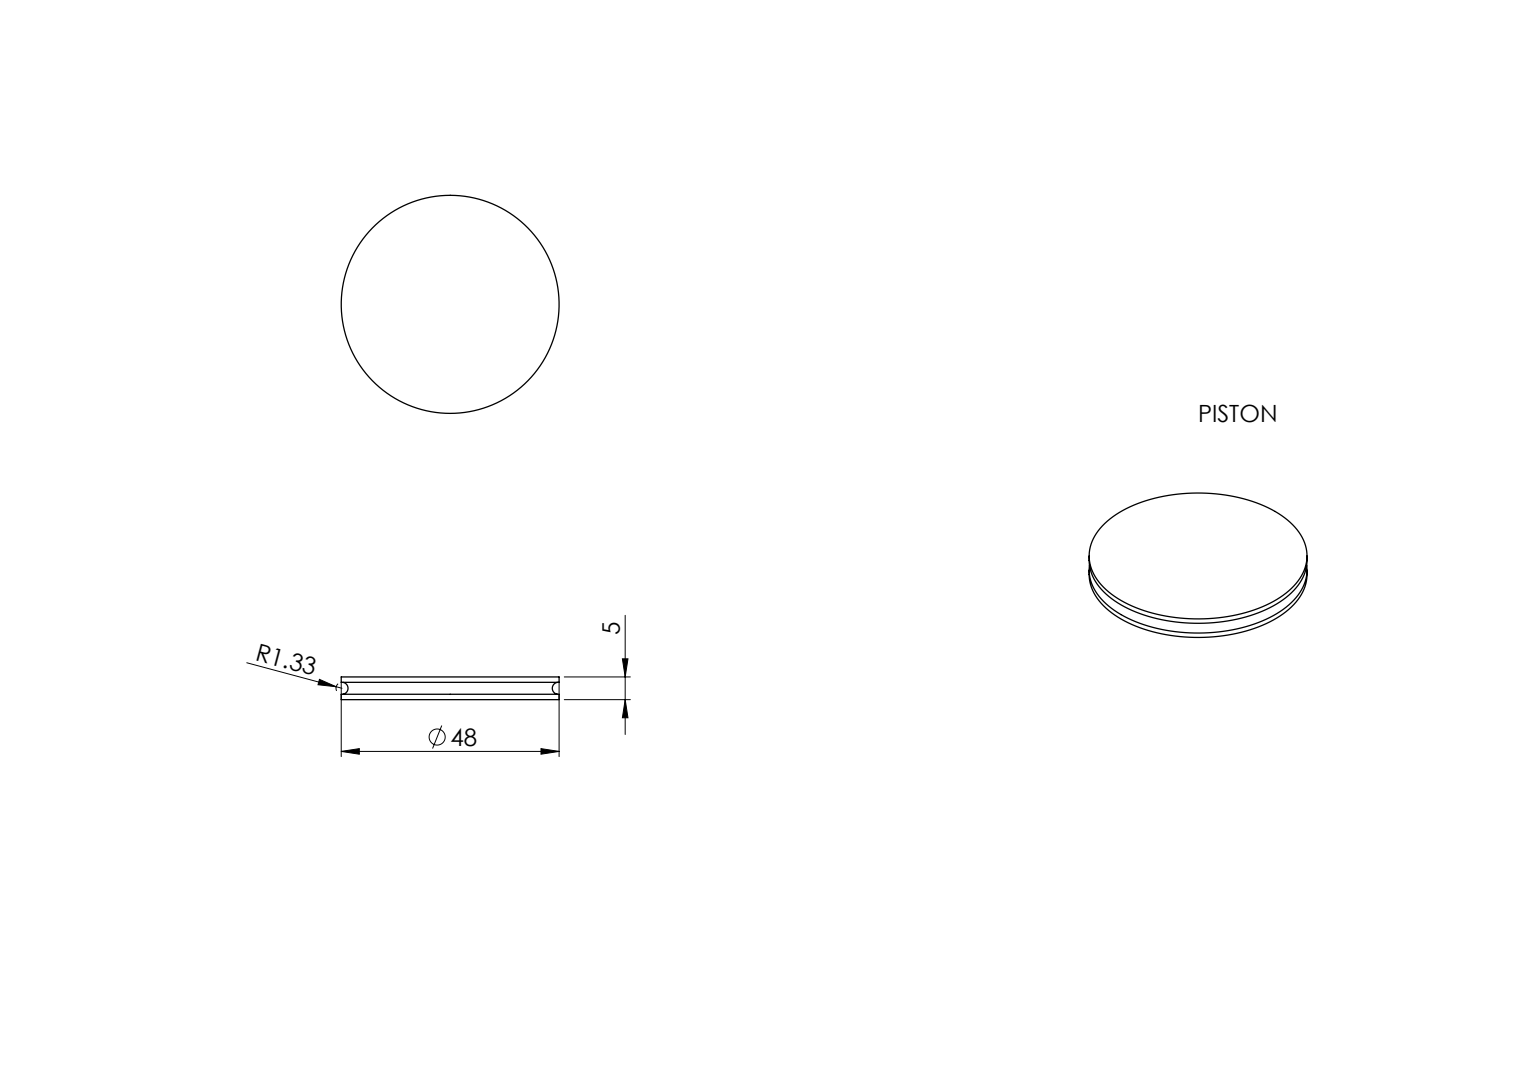
ISO-10303-21;
HEADER;
FILE_DESCRIPTION (('STEP AP214'),
    '1' );
FILE_NAME ('piston.step',
    '2026-10-24T15:06:47',
    ( '' ),
    ( '' ),
    'SwSTEP 2.0',
    'SolidWorks 2026',
    '' );
FILE_SCHEMA (( 'AUTOMOTIVE_DESIGN' ));
ENDSEC;

DATA;
#2=CARTESIAN_POINT ( 'NONE',  ( 0.000000000000000000, 72.50000000000001421, 0.000000000000000000 ) ) ;
#10=FILL_AREA_STYLE_COLOUR ( '', #10270 ) ;
#26=VERTEX_POINT ( 'NONE', #3950 ) ;
#50=AXIS2_PLACEMENT_3D ( 'NONE', #9695, #1591, #1737 ) ;
#62=FILL_AREA_STYLE ('',( #10 ) ) ;
#177=SHAPE_REPRESENTATION ( 'piston', ( #5055 ), #738 ) ;
#247=CARTESIAN_POINT ( 'NONE',  ( 0.000000000000000000, 73.81339255365637086, 0.000000000000000000 ) ) ;
#277=ORIENTED_EDGE ( 'NONE', *, *, #5688, .F. ) ;
#283=DIRECTION ( 'NONE',  ( 8.881784197001252323E-16, 0.000000000000000000, 1.000000000000000000 ) ) ;
#310=EDGE_CURVE ( 'NONE', #1877, #7747, #8787, .T. ) ;
#387=CARTESIAN_POINT ( 'NONE',  ( 2.939152317953647500E-15, 73.81339255365637086, -23.99999999999999645 ) ) ;
#440=AXIS2_PLACEMENT_3D ( 'NONE', #5333, #6948, #1461 ) ;
#452=CARTESIAN_POINT ( 'NONE',  ( 22.50000000000000355, 72.50000000000001421, -2.755455298081545172E-15 ) ) ;
#482=ORIENTED_EDGE ( 'NONE', *, *, #7517, .T. ) ;
#553=ADVANCED_FACE ( 'NONE', ( #6389 ), #3451, .F. ) ;
#580=CIRCLE ( 'NONE', #7259, 23.99999999999999645 ) ;
#600=VERTEX_POINT ( 'NONE', #6490 ) ;
#615=AXIS2_PLACEMENT_3D ( 'NONE', #4071, #9758, #8930 ) ;
#664=DIRECTION ( 'NONE',  ( -0.000000000000000000, 1.000000000000000000, -0.000000000000000000 ) ) ;
#710=FACE_OUTER_BOUND ( 'NONE', #8929, .T. ) ;
#738=( GEOMETRIC_REPRESENTATION_CONTEXT ( 3 ) GLOBAL_UNCERTAINTY_ASSIGNED_CONTEXT ( ( #10215 ) ) GLOBAL_UNIT_ASSIGNED_CONTEXT ( ( #2949, #3785, #10172 ) ) REPRESENTATION_CONTEXT ( 'NONE', 'WORKASPACE' ) );
#753=CIRCLE ( 'NONE', #7274, 23.99999999999999645 ) ;
#782=DIRECTION ( 'NONE',  ( -0.000000000000000000, 1.000000000000000000, -0.000000000000000000 ) ) ;
#784=ADVANCED_FACE ( 'NONE', ( #710 ), #3851, .T. ) ;
#858=EDGE_CURVE ( 'NONE', #7847, #7747, #5465, .T. ) ;
#887=EDGE_CURVE ( 'NONE', #1976, #26, #7608, .T. ) ;
#901=SHAPE_REPRESENTATION_RELATIONSHIP ( 'NONE' , 'NONE' ,  #177, #3150 ) ;
#953=DIRECTION ( 'NONE',  ( 1.000000000000000000, 0.000000000000000000, 0.000000000000000000 ) ) ;
#1070=CARTESIAN_POINT ( 'NONE',  ( 0.000000000000000000, 73.81339255365637086, 0.000000000000000000 ) ) ;
#1076=CARTESIAN_POINT ( 'NONE',  ( -22.50000000000000355, 72.50000000000001421, 0.000000000000000000 ) ) ;
#1138=CIRCLE ( 'NONE', #6996, 23.99999999999999645 ) ;
#1416=UNCERTAINTY_MEASURE_WITH_UNIT (LENGTH_MEASURE( 1.000000000000000082E-05 ), #8634, 'distance_accuracy_value', 'NONE');
#1421=PRODUCT_DEFINITION_SHAPE ( 'NONE', 'NONE',  #3149 ) ;
#1458=( NAMED_UNIT ( * ) PLANE_ANGLE_UNIT ( ) SI_UNIT ( $, .RADIAN. ) );
#1461=DIRECTION ( 'NONE',  ( -1.000000000000000000, 0.000000000000000000, 1.224646799147352961E-16 ) ) ;
#1480=SURFACE_STYLE_FILL_AREA ( #62 ) ;
#1509=ORIENTED_EDGE ( 'NONE', *, *, #310, .F. ) ;
#1546=CARTESIAN_POINT ( 'NONE',  ( 0.000000000000000000, 75.00000000000001421, 0.000000000000000000 ) ) ;
#1550=ORIENTED_EDGE ( 'NONE', *, *, #4131, .T. ) ;
#1570=( GEOMETRIC_REPRESENTATION_CONTEXT ( 3 ) GLOBAL_UNCERTAINTY_ASSIGNED_CONTEXT ( ( #2145 ) ) GLOBAL_UNIT_ASSIGNED_CONTEXT ( ( #2268, #3164, #9494 ) ) REPRESENTATION_CONTEXT ( 'NONE', 'WORKASPACE' ) );
#1591=DIRECTION ( 'NONE',  ( 0.000000000000000000, -1.000000000000000000, 0.000000000000000000 ) ) ;
#1601=LINE ( 'NONE', #7991, #10153 ) ;
#1631=ORIENTED_EDGE ( 'NONE', *, *, #5530, .F. ) ;
#1685=DIRECTION ( 'NONE',  ( 0.000000000000000000, -1.000000000000000000, 0.000000000000000000 ) ) ;
#1737=DIRECTION ( 'NONE',  ( 0.000000000000000000, 0.000000000000000000, -1.000000000000000000 ) ) ;
#1749=ORIENTED_EDGE ( 'NONE', *, *, #5688, .T. ) ;
#1765=EDGE_CURVE ( 'NONE', #8002, #10148, #10057, .T. ) ;
#1877=VERTEX_POINT ( 'NONE', #387 ) ;
#1880=EDGE_CURVE ( 'NONE', #2411, #4835, #5392, .T. ) ;
#1885=ORIENTED_EDGE ( 'NONE', *, *, #7543, .T. ) ;
#1897=EDGE_CURVE ( 'NONE', #4746, #8517, #7219, .T. ) ;
#1957=DIRECTION ( 'NONE',  ( -0.000000000000000000, -1.000000000000000000, 0.000000000000000000 ) ) ;
#1976=VERTEX_POINT ( 'NONE', #2173 ) ;
#2004=DIRECTION ( 'NONE',  ( -1.000000000000000000, 0.000000000000000000, 0.000000000000000000 ) ) ;
#2016=CIRCLE ( 'NONE', #6212, 22.50000000000000355 ) ;
#2040=AXIS2_PLACEMENT_3D ( 'NONE', #2702, #1957, #2004 ) ;
#2057=MECHANICAL_DESIGN_GEOMETRIC_PRESENTATION_REPRESENTATION('',(#9429),#1570);
#2145=UNCERTAINTY_MEASURE_WITH_UNIT (LENGTH_MEASURE( 1.000000000000000082E-05 ), #2268, 'distance_accuracy_value', 'NONE');
#2161=EDGE_LOOP ( 'NONE', ( #1509, #3667, #482, #1885, #5735 ) ) ;
#2173=CARTESIAN_POINT ( 'NONE',  ( -24.00000000000000711, 71.18660744634364335, 0.000000000000000000 ) ) ;
#2196=PRODUCT_CONTEXT ( 'NONE', #7453, 'mechanical' ) ;
#2268=( LENGTH_UNIT ( ) NAMED_UNIT ( * ) SI_UNIT ( .MILLI., .METRE. ) );
#2320=EDGE_CURVE ( 'NONE', #2411, #600, #3373, .T. ) ;
#2345=DIRECTION ( 'NONE',  ( 0.000000000000000000, 0.000000000000000000, 1.000000000000000000 ) ) ;
#2375=ADVANCED_FACE ( 'NONE', ( #4272 ), #5566, .F. ) ;
#2411=VERTEX_POINT ( 'NONE', #1076 ) ;
#2441=AXIS2_PLACEMENT_3D ( 'NONE', #6592, #8319, #953 ) ;
#2478=CARTESIAN_POINT ( 'NONE',  ( 0.000000000000000000, 73.81339255365637086, 0.000000000000000000 ) ) ;
#2562=DIRECTION ( 'NONE',  ( -1.000000000000000000, 0.000000000000000000, 0.000000000000000000 ) ) ;
#2596=TOROIDAL_SURFACE ( 'NONE', #5935, 23.82500000000000284, 1.324999999999999956 ) ;
#2702=CARTESIAN_POINT ( 'NONE',  ( 0.000000000000000000, 72.50000000000001421, 0.000000000000000000 ) ) ;
#2722=CARTESIAN_POINT ( 'NONE',  ( 2.939152317953647500E-15, 70.00000000000000000, -23.99999999999999645 ) ) ;
#2812=DIRECTION ( 'NONE',  ( 0.000000000000000000, 1.000000000000000000, -0.000000000000000000 ) ) ;
#2913=PLANE ( 'NONE',  #8914 ) ;
#2923=EDGE_LOOP ( 'NONE', ( #7895, #6101 ) ) ;
#2949=( LENGTH_UNIT ( ) NAMED_UNIT ( * ) SI_UNIT ( .MILLI., .METRE. ) );
#2987=AXIS2_PLACEMENT_3D ( 'NONE', #2478, #9690, #8908 ) ;
#3019=ORIENTED_EDGE ( 'NONE', *, *, #1880, .F. ) ;
#3075=CARTESIAN_POINT ( 'NONE',  ( 0.000000000000000000, 71.18660744634364335, 0.000000000000000000 ) ) ;
#3129=DIRECTION ( 'NONE',  ( 0.000000000000000000, 0.000000000000000000, 1.000000000000000000 ) ) ;
#3138=DIRECTION ( 'NONE',  ( -1.000000000000000000, 0.000000000000000000, 1.224646799147352961E-16 ) ) ;
#3149=PRODUCT_DEFINITION ( 'UNKNOWN', '', #5131, #9255 ) ;
#3150=ADVANCED_BREP_SHAPE_REPRESENTATION ( '', ( #6259, #5055 ), #738 ) ;
#3164=( NAMED_UNIT ( * ) PLANE_ANGLE_UNIT ( ) SI_UNIT ( $, .RADIAN. ) );
#3235=CIRCLE ( 'NONE', #50, 23.99999999999999645 ) ;
#3253=DIRECTION ( 'NONE',  ( -1.000000000000000000, 0.000000000000000000, 0.000000000000000000 ) ) ;
#3280=CIRCLE ( 'NONE', #9774, 1.324999999999999734 ) ;
#3333=CARTESIAN_POINT ( 'NONE',  ( 0.000000000000000000, 70.00000000000000000, 23.99999999999999645 ) ) ;
#3337=EDGE_CURVE ( 'NONE', #7747, #7847, #3235, .T. ) ;
#3342=FACE_OUTER_BOUND ( 'NONE', #5022, .T. ) ;
#3373=CIRCLE ( 'NONE', #7726, 1.324999999999999734 ) ;
#3385=DIRECTION ( 'NONE',  ( -0.000000000000000000, -1.000000000000000000, 0.000000000000000000 ) ) ;
#3393=ORIENTED_EDGE ( 'NONE', *, *, #3520, .T. ) ;
#3451=TOROIDAL_SURFACE ( 'NONE', #9300, 23.82500000000000284, 1.324999999999999956 ) ;
#3520=EDGE_CURVE ( 'NONE', #4835, #2411, #2016, .T. ) ;
#3524=DIRECTION ( 'NONE',  ( -0.000000000000000000, -1.000000000000000000, 0.000000000000000000 ) ) ;
#3594=AXIS2_PLACEMENT_3D ( 'NONE', #247, #2812, #5797 ) ;
#3599=PLANE ( 'NONE',  #10350 ) ;
#3654=CARTESIAN_POINT ( 'NONE',  ( 0.000000000000000000, 75.00000000000001421, 0.000000000000000000 ) ) ;
#3667=ORIENTED_EDGE ( 'NONE', *, *, #6650, .T. ) ;
#3705=DIRECTION ( 'NONE',  ( 0.000000000000000000, -0.000000000000000000, -1.000000000000000000 ) ) ;
#3733=DIRECTION ( 'NONE',  ( 0.000000000000000000, 0.000000000000000000, 1.000000000000000000 ) ) ;
#3783=AXIS2_PLACEMENT_3D ( 'NONE', #1546, #10130, #10243 ) ;
#3785=( NAMED_UNIT ( * ) PLANE_ANGLE_UNIT ( ) SI_UNIT ( $, .RADIAN. ) );
#3787=DIRECTION ( 'NONE',  ( 0.000000000000000000, 0.000000000000000000, 1.000000000000000000 ) ) ;
#3809=ORIENTED_EDGE ( 'NONE', *, *, #4131, .F. ) ;
#3816=DIRECTION ( 'NONE',  ( -0.000000000000000000, 1.000000000000000000, -0.000000000000000000 ) ) ;
#3851=CYLINDRICAL_SURFACE ( 'NONE', #10131, 23.99999999999999645 ) ;
#3946=VECTOR ( 'NONE', #9820, 1000.000000000000000 ) ;
#3950=CARTESIAN_POINT ( 'NONE',  ( 2.939152317953647500E-15, 71.18660744634364335, -23.99999999999999645 ) ) ;
#3962=TOROIDAL_SURFACE ( 'NONE', #5960, 23.82500000000000284, 1.324999999999999956 ) ;
#3965=CARTESIAN_POINT ( 'NONE',  ( 0.000000000000000000, 72.50000000000001421, 0.000000000000000000 ) ) ;
#4071=CARTESIAN_POINT ( 'NONE',  ( 0.000000000000000000, 70.00000000000000000, 0.000000000000000000 ) ) ;
#4096=CIRCLE ( 'NONE', #8106, 23.99999999999999645 ) ;
#4115=EDGE_CURVE ( 'NONE', #8517, #1976, #580, .T. ) ;
#4131=EDGE_CURVE ( 'NONE', #26, #4746, #4096, .T. ) ;
#4154=DIRECTION ( 'NONE',  ( 0.000000000000000000, 0.000000000000000000, 1.000000000000000000 ) ) ;
#4262=CIRCLE ( 'NONE', #2441, 1.324999999999999734 ) ;
#4264=CYLINDRICAL_SURFACE ( 'NONE', #615, 23.99999999999999645 ) ;
#4272=FACE_OUTER_BOUND ( 'NONE', #6236, .T. ) ;
#4278=CARTESIAN_POINT ( 'NONE',  ( 0.000000000000000000, 72.50000000000001421, 0.000000000000000000 ) ) ;
#4286=CARTESIAN_POINT ( 'NONE',  ( 0.000000000000000000, 73.81339255365637086, 0.000000000000000000 ) ) ;
#4314=DIRECTION ( 'NONE',  ( 0.000000000000000000, 1.000000000000000000, -0.000000000000000000 ) ) ;
#4352=STYLED_ITEM('',(#10394),#6259);
#4369=DIRECTION ( 'NONE',  ( 0.000000000000000000, -0.000000000000000000, -1.000000000000000000 ) ) ;
#4405=EDGE_CURVE ( 'NONE', #6757, #6493, #753, .T. ) ;
#4412=EDGE_LOOP ( 'NONE', ( #6624, #4996, #1550, #5367, #6893 ) ) ;
#4416=DIRECTION ( 'NONE',  ( -0.000000000000000000, -1.000000000000000000, 0.000000000000000000 ) ) ;
#4506=EDGE_LOOP ( 'NONE', ( #9987, #1631, #4846, #6958, #5378 ) ) ;
#4524=FACE_OUTER_BOUND ( 'NONE', #4412, .T. ) ;
#4583=DIRECTION ( 'NONE',  ( 0.000000000000000000, 0.000000000000000000, 1.000000000000000000 ) ) ;
#4622=CARTESIAN_POINT ( 'NONE',  ( 0.000000000000000000, 71.18660744634364335, 0.000000000000000000 ) ) ;
#4650=CYLINDRICAL_SURFACE ( 'NONE', #9705, 23.99999999999999645 ) ;
#4746=VERTEX_POINT ( 'NONE', #9036 ) ;
#4749=DIRECTION ( 'NONE',  ( -1.224646799147353207E-16, 0.000000000000000000, -1.000000000000000000 ) ) ;
#4835=VERTEX_POINT ( 'NONE', #452 ) ;
#4846=ORIENTED_EDGE ( 'NONE', *, *, #5943, .T. ) ;
#4951=AXIS2_PLACEMENT_3D ( 'NONE', #7719, #5987, #4583 ) ;
#4996=ORIENTED_EDGE ( 'NONE', *, *, #8566, .T. ) ;
#5022=EDGE_LOOP ( 'NONE', ( #1749, #6205, #6376, #3809, #9862 ) ) ;
#5055=AXIS2_PLACEMENT_3D ( 'NONE', #9842, #4154, #9744 ) ;
#5079=ORIENTED_EDGE ( 'NONE', *, *, #7948, .F. ) ;
#5131=PRODUCT_DEFINITION_FORMATION_WITH_SPECIFIED_SOURCE ( 'ANY', '', #5693, .NOT_KNOWN. ) ;
#5203=AXIS2_PLACEMENT_3D ( 'NONE', #4286, #6741, #7470 ) ;
#5251=EDGE_LOOP ( 'NONE', ( #3019, #9847, #8245, #8860, #5079 ) ) ;
#5252=CARTESIAN_POINT ( 'NONE',  ( 2.939152317953647500E-15, 75.00000000000001421, -23.99999999999999645 ) ) ;
#5311=EDGE_CURVE ( 'NONE', #10148, #1877, #7113, .T. ) ;
#5333=CARTESIAN_POINT ( 'NONE',  ( 23.82500000000000284, 72.50000000000001421, -2.917720998968569322E-15 ) ) ;
#5367=ORIENTED_EDGE ( 'NONE', *, *, #1897, .T. ) ;
#5378=ORIENTED_EDGE ( 'NONE', *, *, #887, .T. ) ;
#5392=CIRCLE ( 'NONE', #6553, 22.50000000000000355 ) ;
#5401=ORIENTED_EDGE ( 'NONE', *, *, #2320, .F. ) ;
#5465=CIRCLE ( 'NONE', #3783, 23.99999999999999645 ) ;
#5467=PRESENTATION_STYLE_ASSIGNMENT (( #9638 ) ) ;
#5468=DIRECTION ( 'NONE',  ( -0.000000000000000000, -1.000000000000000000, 0.000000000000000000 ) ) ;
#5491=EDGE_CURVE ( 'NONE', #4746, #4835, #3280, .T. ) ;
#5519=CARTESIAN_POINT ( 'NONE',  ( 0.000000000000000000, 70.00000000000000000, 0.000000000000000000 ) ) ;
#5530=EDGE_CURVE ( 'NONE', #6493, #6757, #10126, .T. ) ;
#5564=SURFACE_SIDE_STYLE ('',( #1480 ) ) ;
#5566=TOROIDAL_SURFACE ( 'NONE', #2040, 23.82500000000000284, 1.324999999999999956 ) ;
#5642=VECTOR ( 'NONE', #782, 1000.000000000000000 ) ;
#5644=DIRECTION ( 'NONE',  ( 0.000000000000000000, -1.000000000000000000, 0.000000000000000000 ) ) ;
#5688=EDGE_CURVE ( 'NONE', #1976, #2411, #4262, .T. ) ;
#5693=PRODUCT ( 'piston', 'piston', '', ( #2196 ) ) ;
#5694=ORIENTED_EDGE ( 'NONE', *, *, #4115, .F. ) ;
#5735=ORIENTED_EDGE ( 'NONE', *, *, #858, .T. ) ;
#5797=DIRECTION ( 'NONE',  ( -8.881784197001252323E-16, 0.000000000000000000, -1.000000000000000000 ) ) ;
#5852=MECHANICAL_DESIGN_GEOMETRIC_PRESENTATION_REPRESENTATION('',(#4352),#7037);
#5933=ADVANCED_FACE ( 'NONE', ( #3342 ), #2596, .F. ) ;
#5935=AXIS2_PLACEMENT_3D ( 'NONE', #4278, #3385, #2562 ) ;
#5943=EDGE_CURVE ( 'NONE', #6493, #8517, #9040, .T. ) ;
#5960=AXIS2_PLACEMENT_3D ( 'NONE', #6197, #8444, #10185 ) ;
#5987=DIRECTION ( 'NONE',  ( -0.000000000000000000, 1.000000000000000000, -0.000000000000000000 ) ) ;
#6023=ORIENTED_EDGE ( 'NONE', *, *, #5530, .T. ) ;
#6094=CYLINDRICAL_SURFACE ( 'NONE', #4951, 23.99999999999999645 ) ;
#6096=DIRECTION ( 'NONE',  ( 0.000000000000000000, -1.000000000000000000, 0.000000000000000000 ) ) ;
#6101=ORIENTED_EDGE ( 'NONE', *, *, #3337, .F. ) ;
#6157=VECTOR ( 'NONE', #9808, 1000.000000000000000 ) ;
#6191=CARTESIAN_POINT ( 'NONE',  ( 0.000000000000000000, 70.00000000000000000, 23.99999999999999645 ) ) ;
#6197=CARTESIAN_POINT ( 'NONE',  ( 0.000000000000000000, 72.50000000000001421, 0.000000000000000000 ) ) ;
#6205=ORIENTED_EDGE ( 'NONE', *, *, #1880, .T. ) ;
#6212=AXIS2_PLACEMENT_3D ( 'NONE', #3965, #7151, #9564 ) ;
#6236=EDGE_LOOP ( 'NONE', ( #6658, #9594, #10061, #8627, #5401 ) ) ;
#6259=MANIFOLD_SOLID_BREP ( 'Cavity1', #10150 ) ;
#6269=ADVANCED_FACE ( 'NONE', ( #6426 ), #4650, .T. ) ;
#6376=ORIENTED_EDGE ( 'NONE', *, *, #5491, .F. ) ;
#6389=FACE_OUTER_BOUND ( 'NONE', #5251, .T. ) ;
#6413=ADVANCED_FACE ( 'NONE', ( #9080 ), #4264, .T. ) ;
#6426=FACE_OUTER_BOUND ( 'NONE', #2161, .T. ) ;
#6490=CARTESIAN_POINT ( 'NONE',  ( -24.00000000000000711, 73.81339255365637086, 0.000000000000000000 ) ) ;
#6493=VERTEX_POINT ( 'NONE', #6191 ) ;
#6540=ORIENTED_EDGE ( 'NONE', *, *, #1765, .T. ) ;
#6553=AXIS2_PLACEMENT_3D ( 'NONE', #7601, #3524, #7441 ) ;
#6592=CARTESIAN_POINT ( 'NONE',  ( -23.82500000000000284, 72.50000000000001421, 0.000000000000000000 ) ) ;
#6624=ORIENTED_EDGE ( 'NONE', *, *, #4405, .F. ) ;
#6650=EDGE_CURVE ( 'NONE', #1877, #600, #7475, .T. ) ;
#6658=ORIENTED_EDGE ( 'NONE', *, *, #3520, .F. ) ;
#6741=DIRECTION ( 'NONE',  ( 0.000000000000000000, 1.000000000000000000, -0.000000000000000000 ) ) ;
#6757=VERTEX_POINT ( 'NONE', #2722 ) ;
#6770=ORIENTED_EDGE ( 'NONE', *, *, #310, .T. ) ;
#6826=DIRECTION ( 'NONE',  ( 1.000000000000000000, 0.000000000000000000, 0.000000000000000000 ) ) ;
#6834=DIRECTION ( 'NONE',  ( 0.000000000000000000, -1.000000000000000000, 0.000000000000000000 ) ) ;
#6893=ORIENTED_EDGE ( 'NONE', *, *, #5943, .F. ) ;
#6895=SHAPE_DEFINITION_REPRESENTATION ( #1421, #177 ) ;
#6911=EDGE_LOOP ( 'NONE', ( #6023, #9540 ) ) ;
#6948=DIRECTION ( 'NONE',  ( -1.224646799147353207E-16, 0.000000000000000000, -1.000000000000000000 ) ) ;
#6958=ORIENTED_EDGE ( 'NONE', *, *, #4115, .T. ) ;
#6996=AXIS2_PLACEMENT_3D ( 'NONE', #1070, #4314, #8981 ) ;
#7037=( GEOMETRIC_REPRESENTATION_CONTEXT ( 3 ) GLOBAL_UNCERTAINTY_ASSIGNED_CONTEXT ( ( #1416 ) ) GLOBAL_UNIT_ASSIGNED_CONTEXT ( ( #8634, #1458, #7842 ) ) REPRESENTATION_CONTEXT ( 'NONE', 'WORKASPACE' ) );
#7113=CIRCLE ( 'NONE', #3594, 23.99999999999999645 ) ;
#7121=DIRECTION ( 'NONE',  ( -0.000000000000000000, -1.000000000000000000, 0.000000000000000000 ) ) ;
#7151=DIRECTION ( 'NONE',  ( -0.000000000000000000, -1.000000000000000000, 0.000000000000000000 ) ) ;
#7155=DIRECTION ( 'NONE',  ( 0.000000000000000000, 0.000000000000000000, -1.000000000000000000 ) ) ;
#7219=CIRCLE ( 'NONE', #8898, 23.99999999999999645 ) ;
#7257=ORIENTED_EDGE ( 'NONE', *, *, #5311, .T. ) ;
#7259=AXIS2_PLACEMENT_3D ( 'NONE', #4622, #8658, #3787 ) ;
#7274=AXIS2_PLACEMENT_3D ( 'NONE', #5519, #1685, #8072 ) ;
#7286=AXIS2_PLACEMENT_3D ( 'NONE', #3075, #9401, #8621 ) ;
#7339=ADVANCED_FACE ( 'NONE', ( #7732 ), #3599, .F. ) ;
#7441=DIRECTION ( 'NONE',  ( 0.000000000000000000, 0.000000000000000000, -1.000000000000000000 ) ) ;
#7453=APPLICATION_CONTEXT ( 'automotive_design' ) ;
#7470=DIRECTION ( 'NONE',  ( 0.000000000000000000, 0.000000000000000000, -1.000000000000000000 ) ) ;
#7475=CIRCLE ( 'NONE', #2987, 23.99999999999999645 ) ;
#7517=EDGE_CURVE ( 'NONE', #600, #8002, #1138, .T. ) ;
#7543=EDGE_CURVE ( 'NONE', #8002, #7847, #9759, .T. ) ;
#7601=CARTESIAN_POINT ( 'NONE',  ( 0.000000000000000000, 72.50000000000001421, 0.000000000000000000 ) ) ;
#7608=CIRCLE ( 'NONE', #7286, 23.99999999999999645 ) ;
#7719=CARTESIAN_POINT ( 'NONE',  ( 0.000000000000000000, 70.00000000000000000, 0.000000000000000000 ) ) ;
#7726=AXIS2_PLACEMENT_3D ( 'NONE', #8298, #9920, #6826 ) ;
#7732=FACE_OUTER_BOUND ( 'NONE', #2923, .T. ) ;
#7747=VERTEX_POINT ( 'NONE', #5252 ) ;
#7842=( NAMED_UNIT ( * ) SI_UNIT ( $, .STERADIAN. ) SOLID_ANGLE_UNIT ( ) );
#7847=VERTEX_POINT ( 'NONE', #8307 ) ;
#7895=ORIENTED_EDGE ( 'NONE', *, *, #858, .F. ) ;
#7948=EDGE_CURVE ( 'NONE', #4835, #10148, #9302, .T. ) ;
#7951=CARTESIAN_POINT ( 'NONE',  ( 2.939152317953647500E-15, 70.00000000000000000, -23.99999999999999645 ) ) ;
#7976=ORIENTED_EDGE ( 'NONE', *, *, #1897, .F. ) ;
#7991=CARTESIAN_POINT ( 'NONE',  ( 2.939152317953647500E-15, 70.00000000000000000, -23.99999999999999645 ) ) ;
#8002=VERTEX_POINT ( 'NONE', #10032 ) ;
#8046=CARTESIAN_POINT ( 'NONE',  ( 0.000000000000000000, 70.00000000000000000, 0.000000000000000000 ) ) ;
#8072=DIRECTION ( 'NONE',  ( 0.000000000000000000, 0.000000000000000000, -1.000000000000000000 ) ) ;
#8106=AXIS2_PLACEMENT_3D ( 'NONE', #10055, #5468, #3733 ) ;
#8245=ORIENTED_EDGE ( 'NONE', *, *, #6650, .F. ) ;
#8278=AXIS2_PLACEMENT_3D ( 'NONE', #8046, #5644, #7155 ) ;
#8298=CARTESIAN_POINT ( 'NONE',  ( -23.82500000000000284, 72.50000000000001421, 0.000000000000000000 ) ) ;
#8307=CARTESIAN_POINT ( 'NONE',  ( 0.000000000000000000, 75.00000000000001421, 23.99999999999999645 ) ) ;
#8319=DIRECTION ( 'NONE',  ( 0.000000000000000000, 0.000000000000000000, 1.000000000000000000 ) ) ;
#8378=ADVANCED_FACE ( 'NONE', ( #4524 ), #6094, .T. ) ;
#8444=DIRECTION ( 'NONE',  ( -0.000000000000000000, -1.000000000000000000, 0.000000000000000000 ) ) ;
#8517=VERTEX_POINT ( 'NONE', #10352 ) ;
#8548=APPLICATION_CONTEXT ( 'automotive_design' ) ;
#8566=EDGE_CURVE ( 'NONE', #6757, #26, #1601, .T. ) ;
#8621=DIRECTION ( 'NONE',  ( 0.000000000000000000, 0.000000000000000000, 1.000000000000000000 ) ) ;
#8627=ORIENTED_EDGE ( 'NONE', *, *, #7517, .F. ) ;
#8634=( LENGTH_UNIT ( ) NAMED_UNIT ( * ) SI_UNIT ( .MILLI., .METRE. ) );
#8658=DIRECTION ( 'NONE',  ( -0.000000000000000000, -1.000000000000000000, 0.000000000000000000 ) ) ;
#8681=ORIENTED_EDGE ( 'NONE', *, *, #5491, .T. ) ;
#8787=LINE ( 'NONE', #7951, #5642 ) ;
#8860=ORIENTED_EDGE ( 'NONE', *, *, #5311, .F. ) ;
#8898=AXIS2_PLACEMENT_3D ( 'NONE', #9963, #4416, #283 ) ;
#8908=DIRECTION ( 'NONE',  ( 0.000000000000000000, 0.000000000000000000, -1.000000000000000000 ) ) ;
#8914=AXIS2_PLACEMENT_3D ( 'NONE', #10021, #6096, #4369 ) ;
#8926=FACE_OUTER_BOUND ( 'NONE', #9903, .T. ) ;
#8929=EDGE_LOOP ( 'NONE', ( #7257, #6770, #8948, #9224, #6540 ) ) ;
#8930=DIRECTION ( 'NONE',  ( 0.000000000000000000, 0.000000000000000000, 1.000000000000000000 ) ) ;
#8948=ORIENTED_EDGE ( 'NONE', *, *, #3337, .T. ) ;
#8981=DIRECTION ( 'NONE',  ( 0.000000000000000000, 0.000000000000000000, -1.000000000000000000 ) ) ;
#9036=CARTESIAN_POINT ( 'NONE',  ( 24.00000000000000711, 71.18660744634364335, -2.939152317953649078E-15 ) ) ;
#9040=LINE ( 'NONE', #9871, #3946 ) ;
#9080=FACE_OUTER_BOUND ( 'NONE', #4506, .T. ) ;
#9224=ORIENTED_EDGE ( 'NONE', *, *, #7543, .F. ) ;
#9255=PRODUCT_DEFINITION_CONTEXT ( 'detailed design', #8548, 'design' ) ;
#9289=CARTESIAN_POINT ( 'NONE',  ( 24.00000000000000711, 73.81339255365637086, -2.939152317953649078E-15 ) ) ;
#9300=AXIS2_PLACEMENT_3D ( 'NONE', #2, #7121, #3253 ) ;
#9302=CIRCLE ( 'NONE', #440, 1.324999999999999734 ) ;
#9401=DIRECTION ( 'NONE',  ( -0.000000000000000000, -1.000000000000000000, 0.000000000000000000 ) ) ;
#9413=CARTESIAN_POINT ( 'NONE',  ( 0.000000000000000000, 70.00000000000000000, 0.000000000000000000 ) ) ;
#9429=STYLED_ITEM ( 'NONE', ( #5467 ), #3150 ) ;
#9494=( NAMED_UNIT ( * ) SI_UNIT ( $, .STERADIAN. ) SOLID_ANGLE_UNIT ( ) );
#9540=ORIENTED_EDGE ( 'NONE', *, *, #4405, .T. ) ;
#9554=ADVANCED_FACE ( 'NONE', ( #8926 ), #3962, .F. ) ;
#9559=CARTESIAN_POINT ( 'NONE',  ( 0.000000000000000000, 70.00000000000000000, 0.000000000000000000 ) ) ;
#9564=DIRECTION ( 'NONE',  ( 0.000000000000000000, 0.000000000000000000, -1.000000000000000000 ) ) ;
#9594=ORIENTED_EDGE ( 'NONE', *, *, #7948, .T. ) ;
#9638=SURFACE_STYLE_USAGE ( .BOTH. , #5564 ) ;
#9690=DIRECTION ( 'NONE',  ( 0.000000000000000000, 1.000000000000000000, -0.000000000000000000 ) ) ;
#9695=CARTESIAN_POINT ( 'NONE',  ( 0.000000000000000000, 75.00000000000001421, 0.000000000000000000 ) ) ;
#9705=AXIS2_PLACEMENT_3D ( 'NONE', #9413, #3816, #2345 ) ;
#9744=DIRECTION ( 'NONE',  ( 1.000000000000000000, 0.000000000000000000, 0.000000000000000000 ) ) ;
#9758=DIRECTION ( 'NONE',  ( -0.000000000000000000, 1.000000000000000000, -0.000000000000000000 ) ) ;
#9759=LINE ( 'NONE', #3333, #6157 ) ;
#9774=AXIS2_PLACEMENT_3D ( 'NONE', #10305, #4749, #3138 ) ;
#9808=DIRECTION ( 'NONE',  ( -0.000000000000000000, 1.000000000000000000, -0.000000000000000000 ) ) ;
#9820=DIRECTION ( 'NONE',  ( -0.000000000000000000, 1.000000000000000000, -0.000000000000000000 ) ) ;
#9842=CARTESIAN_POINT ( 'NONE',  ( 0.000000000000000000, 0.000000000000000000, 0.000000000000000000 ) ) ;
#9847=ORIENTED_EDGE ( 'NONE', *, *, #2320, .T. ) ;
#9862=ORIENTED_EDGE ( 'NONE', *, *, #887, .F. ) ;
#9871=CARTESIAN_POINT ( 'NONE',  ( 0.000000000000000000, 70.00000000000000000, 23.99999999999999645 ) ) ;
#9903=EDGE_LOOP ( 'NONE', ( #8681, #3393, #277, #5694, #7976 ) ) ;
#9920=DIRECTION ( 'NONE',  ( 0.000000000000000000, 0.000000000000000000, 1.000000000000000000 ) ) ;
#9963=CARTESIAN_POINT ( 'NONE',  ( 0.000000000000000000, 71.18660744634364335, 0.000000000000000000 ) ) ;
#9987=ORIENTED_EDGE ( 'NONE', *, *, #8566, .F. ) ;
#10021=CARTESIAN_POINT ( 'NONE',  ( 0.000000000000000000, 70.00000000000000000, 0.000000000000000000 ) ) ;
#10032=CARTESIAN_POINT ( 'NONE',  ( 0.000000000000000000, 73.81339255365637086, 23.99999999999999645 ) ) ;
#10055=CARTESIAN_POINT ( 'NONE',  ( 0.000000000000000000, 71.18660744634364335, 0.000000000000000000 ) ) ;
#10057=CIRCLE ( 'NONE', #5203, 23.99999999999999645 ) ;
#10061=ORIENTED_EDGE ( 'NONE', *, *, #1765, .F. ) ;
#10076=FACE_OUTER_BOUND ( 'NONE', #6911, .T. ) ;
#10113=ADVANCED_FACE ( 'NONE', ( #10076 ), #2913, .T. ) ;
#10126=CIRCLE ( 'NONE', #8278, 23.99999999999999645 ) ;
#10130=DIRECTION ( 'NONE',  ( 0.000000000000000000, -1.000000000000000000, 0.000000000000000000 ) ) ;
#10131=AXIS2_PLACEMENT_3D ( 'NONE', #9559, #10296, #3129 ) ;
#10148=VERTEX_POINT ( 'NONE', #9289 ) ;
#10150=CLOSED_SHELL ( 'NONE', ( #5933, #9554, #784, #2375, #8378, #6413, #10113, #553, #7339, #6269 ) ) ;
#10153=VECTOR ( 'NONE', #664, 1000.000000000000000 ) ;
#10172=( NAMED_UNIT ( * ) SI_UNIT ( $, .STERADIAN. ) SOLID_ANGLE_UNIT ( ) );
#10185=DIRECTION ( 'NONE',  ( -1.000000000000000000, 0.000000000000000000, 0.000000000000000000 ) ) ;
#10215=UNCERTAINTY_MEASURE_WITH_UNIT (LENGTH_MEASURE( 1.000000000000000082E-05 ), #2949, 'distance_accuracy_value', 'NONE');
#10243=DIRECTION ( 'NONE',  ( 0.000000000000000000, 0.000000000000000000, -1.000000000000000000 ) ) ;
#10270=COLOUR_RGB ( '',0.8941176470588234615, 0.8941176470588234615, 0.8941176470588234615 ) ;
#10296=DIRECTION ( 'NONE',  ( -0.000000000000000000, 1.000000000000000000, -0.000000000000000000 ) ) ;
#10305=CARTESIAN_POINT ( 'NONE',  ( 23.82500000000000284, 72.50000000000001421, -2.917720998968569322E-15 ) ) ;
#10350=AXIS2_PLACEMENT_3D ( 'NONE', #3654, #6834, #3705 ) ;
#10352=CARTESIAN_POINT ( 'NONE',  ( 0.000000000000000000, 71.18660744634364335, 23.99999999999999645 ) ) ;
#10388=COLOUR_RGB('Sky Blue',0.24,0.69,0.87);
#10389=FILL_AREA_STYLE_COLOUR('',#10388);
#10390=FILL_AREA_STYLE('',(#10389));
#10391=SURFACE_STYLE_FILL_AREA(#10390);
#10392=SURFACE_SIDE_STYLE('',(#10391));
#10393=SURFACE_STYLE_USAGE(.BOTH.,#10392);
#10394=PRESENTATION_STYLE_ASSIGNMENT((#10393));
ENDSEC;
END-ISO-10303-21;
